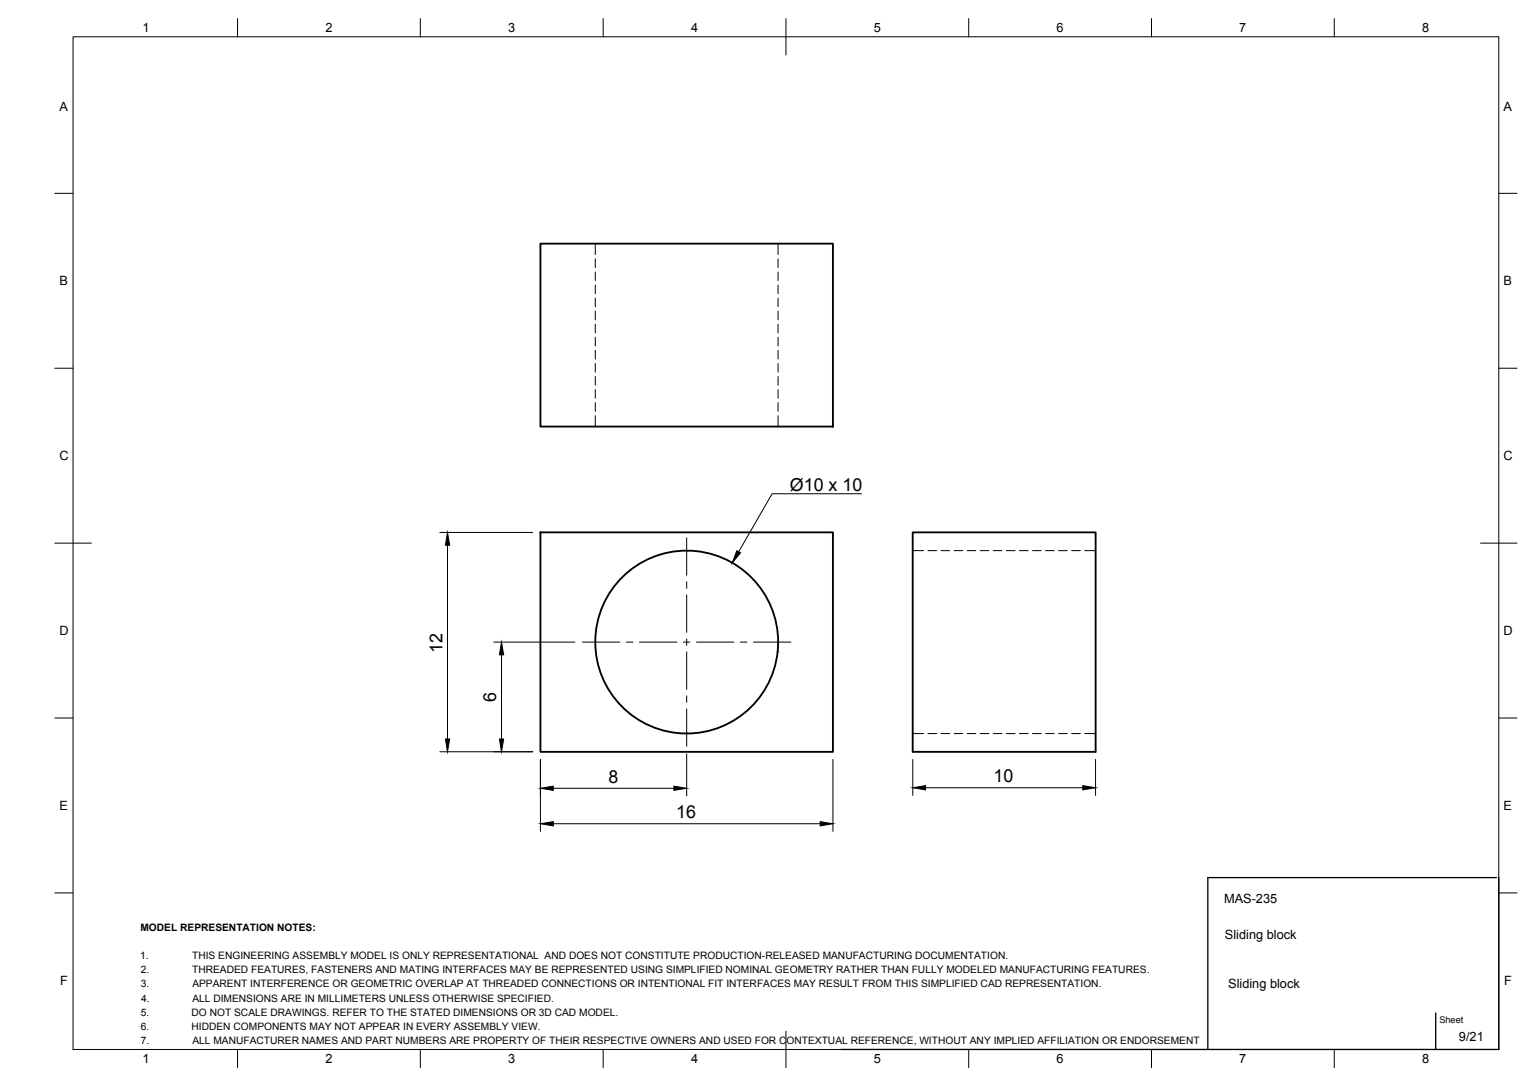
ISO-10303-21;
HEADER;
/* Generated by software containing ST-Developer
 * from STEP Tools, Inc. (www.steptools.com) 
 */

FILE_DESCRIPTION(
/* description */ ('Independent Whitworth quick-return mechanism. Crank radius40, ground-
center spacing80, lever180, connecting rod160, output guide X200. Nomi
nal stroke180 and long/short phase ratio2. Retained guide rods, replac
eable bearing sleeves and captured sliding shoe. No load or production
 rating assigned.'),
/* implementation_level */ '2;1');

FILE_NAME(
/* name */ 'Sliding block.step',
/* time_stamp */ '2026-11-09T18:22:56-08:00',
/* author */ (''),
/* organization */ (''),
/* preprocessor_version */ 'ST-DEVELOPER v20.2',
/* originating_system */ 'Autodesk Translation Framework v15.17.0.0',
/* authorisation */ '');

FILE_SCHEMA (('AUTOMOTIVE_DESIGN { 1 0 10303 214 3 1 1 }'));
ENDSEC;

DATA;
#10=MECHANICAL_DESIGN_GEOMETRIC_PRESENTATION_REPRESENTATION('',(#225),#4388);
#185=SHAPE_REPRESENTATION_RELATIONSHIP('SRR','None',#4484,#205);
#205=ADVANCED_BREP_SHAPE_REPRESENTATION('',(#245),#4374);
#225=STYLED_ITEM('',(#4592),#245);
#245=MANIFOLD_SOLID_BREP('Body1',#2330);
#281=FACE_BOUND('',#624,.T.);
#282=FACE_BOUND('',#626,.T.);
#343=PLANE('',#2660);
#344=PLANE('',#2661);
#345=PLANE('',#2662);
#346=PLANE('',#2663);
#347=PLANE('',#2664);
#348=PLANE('',#2665);
#449=FACE_OUTER_BOUND('',#618,.T.);
#450=FACE_OUTER_BOUND('',#619,.T.);
#451=FACE_OUTER_BOUND('',#620,.T.);
#452=FACE_OUTER_BOUND('',#621,.T.);
#453=FACE_OUTER_BOUND('',#622,.T.);
#454=FACE_OUTER_BOUND('',#623,.T.);
#455=FACE_OUTER_BOUND('',#625,.T.);
#618=EDGE_LOOP('',(#1786,#1787,#1788,#1789));
#619=EDGE_LOOP('',(#1790,#1791,#1792,#1793));
#620=EDGE_LOOP('',(#1794,#1795,#1796,#1797));
#621=EDGE_LOOP('',(#1798,#1799,#1800,#1801));
#622=EDGE_LOOP('',(#1802,#1803,#1804,#1805));
#623=EDGE_LOOP('',(#1806,#1807,#1808,#1809));
#624=EDGE_LOOP('',(#1810));
#625=EDGE_LOOP('',(#1811,#1812,#1813,#1814));
#626=EDGE_LOOP('',(#1815));
#815=LINE('',#3916,#954);
#816=LINE('',#3921,#955);
#817=LINE('',#3923,#956);
#818=LINE('',#3925,#957);
#819=LINE('',#3926,#958);
#820=LINE('',#3929,#959);
#821=LINE('',#3931,#960);
#822=LINE('',#3932,#961);
#823=LINE('',#3935,#962);
#824=LINE('',#3937,#963);
#825=LINE('',#3938,#964);
#826=LINE('',#3940,#965);
#827=LINE('',#3941,#966);
#954=VECTOR('',#3141,5.);
#955=VECTOR('',#3146,10.);
#956=VECTOR('',#3147,10.);
#957=VECTOR('',#3148,10.);
#958=VECTOR('',#3149,10.);
#959=VECTOR('',#3152,10.);
#960=VECTOR('',#3153,10.);
#961=VECTOR('',#3154,10.);
#962=VECTOR('',#3157,10.);
#963=VECTOR('',#3158,10.);
#964=VECTOR('',#3159,10.);
#965=VECTOR('',#3162,10.);
#966=VECTOR('',#3163,10.);
#1077=CIRCLE('',#2658,5.);
#1078=CIRCLE('',#2659,5.);
#1223=VERTEX_POINT('',#3913);
#1224=VERTEX_POINT('',#3915);
#1225=VERTEX_POINT('',#3919);
#1226=VERTEX_POINT('',#3920);
#1227=VERTEX_POINT('',#3922);
#1228=VERTEX_POINT('',#3924);
#1229=VERTEX_POINT('',#3928);
#1230=VERTEX_POINT('',#3930);
#1231=VERTEX_POINT('',#3934);
#1232=VERTEX_POINT('',#3936);
#1429=EDGE_CURVE('',#1223,#1223,#1077,.T.);
#1430=EDGE_CURVE('',#1223,#1224,#815,.T.);
#1431=EDGE_CURVE('',#1224,#1224,#1078,.T.);
#1432=EDGE_CURVE('',#1225,#1226,#816,.T.);
#1433=EDGE_CURVE('',#1226,#1227,#817,.T.);
#1434=EDGE_CURVE('',#1228,#1227,#818,.T.);
#1435=EDGE_CURVE('',#1225,#1228,#819,.T.);
#1436=EDGE_CURVE('',#1229,#1225,#820,.T.);
#1437=EDGE_CURVE('',#1230,#1228,#821,.T.);
#1438=EDGE_CURVE('',#1229,#1230,#822,.T.);
#1439=EDGE_CURVE('',#1231,#1229,#823,.T.);
#1440=EDGE_CURVE('',#1232,#1230,#824,.T.);
#1441=EDGE_CURVE('',#1231,#1232,#825,.T.);
#1442=EDGE_CURVE('',#1226,#1231,#826,.T.);
#1443=EDGE_CURVE('',#1227,#1232,#827,.T.);
#1786=ORIENTED_EDGE('',*,*,#1429,.F.);
#1787=ORIENTED_EDGE('',*,*,#1430,.T.);
#1788=ORIENTED_EDGE('',*,*,#1431,.F.);
#1789=ORIENTED_EDGE('',*,*,#1430,.F.);
#1790=ORIENTED_EDGE('',*,*,#1432,.T.);
#1791=ORIENTED_EDGE('',*,*,#1433,.T.);
#1792=ORIENTED_EDGE('',*,*,#1434,.F.);
#1793=ORIENTED_EDGE('',*,*,#1435,.F.);
#1794=ORIENTED_EDGE('',*,*,#1436,.T.);
#1795=ORIENTED_EDGE('',*,*,#1435,.T.);
#1796=ORIENTED_EDGE('',*,*,#1437,.F.);
#1797=ORIENTED_EDGE('',*,*,#1438,.F.);
#1798=ORIENTED_EDGE('',*,*,#1439,.T.);
#1799=ORIENTED_EDGE('',*,*,#1438,.T.);
#1800=ORIENTED_EDGE('',*,*,#1440,.F.);
#1801=ORIENTED_EDGE('',*,*,#1441,.F.);
#1802=ORIENTED_EDGE('',*,*,#1442,.T.);
#1803=ORIENTED_EDGE('',*,*,#1441,.T.);
#1804=ORIENTED_EDGE('',*,*,#1443,.F.);
#1805=ORIENTED_EDGE('',*,*,#1433,.F.);
#1806=ORIENTED_EDGE('',*,*,#1443,.T.);
#1807=ORIENTED_EDGE('',*,*,#1440,.T.);
#1808=ORIENTED_EDGE('',*,*,#1437,.T.);
#1809=ORIENTED_EDGE('',*,*,#1434,.T.);
#1810=ORIENTED_EDGE('',*,*,#1429,.T.);
#1811=ORIENTED_EDGE('',*,*,#1442,.F.);
#1812=ORIENTED_EDGE('',*,*,#1432,.F.);
#1813=ORIENTED_EDGE('',*,*,#1436,.F.);
#1814=ORIENTED_EDGE('',*,*,#1439,.F.);
#1815=ORIENTED_EDGE('',*,*,#1431,.T.);
#2136=CYLINDRICAL_SURFACE('',#2657,5.);
#2221=ADVANCED_FACE('',(#449),#2136,.F.);
#2222=ADVANCED_FACE('',(#450),#343,.T.);
#2223=ADVANCED_FACE('',(#451),#344,.T.);
#2224=ADVANCED_FACE('',(#452),#345,.T.);
#2225=ADVANCED_FACE('',(#453),#346,.T.);
#2226=ADVANCED_FACE('',(#454,#281),#347,.T.);
#2227=ADVANCED_FACE('',(#455,#282),#348,.F.);
#2330=CLOSED_SHELL('',(#2221,#2222,#2223,#2224,#2225,#2226,#2227));
#2656=AXIS2_PLACEMENT_3D('',#3911,#3135,#3136);
#2657=AXIS2_PLACEMENT_3D('',#3912,#3137,#3138);
#2658=AXIS2_PLACEMENT_3D('',#3914,#3139,#3140);
#2659=AXIS2_PLACEMENT_3D('',#3917,#3142,#3143);
#2660=AXIS2_PLACEMENT_3D('',#3918,#3144,#3145);
#2661=AXIS2_PLACEMENT_3D('',#3927,#3150,#3151);
#2662=AXIS2_PLACEMENT_3D('',#3933,#3155,#3156);
#2663=AXIS2_PLACEMENT_3D('',#3939,#3160,#3161);
#2664=AXIS2_PLACEMENT_3D('',#3942,#3164,#3165);
#2665=AXIS2_PLACEMENT_3D('',#3943,#3166,#3167);
#3135=DIRECTION('axis',(0.,0.,1.));
#3136=DIRECTION('refdir',(1.,0.,0.));
#3137=DIRECTION('center_axis',(0.,0.,-1.));
#3138=DIRECTION('ref_axis',(1.,0.,0.));
#3139=DIRECTION('center_axis',(0.,0.,-1.));
#3140=DIRECTION('ref_axis',(1.,0.,0.));
#3141=DIRECTION('',(0.,0.,-1.));
#3142=DIRECTION('center_axis',(0.,0.,1.));
#3143=DIRECTION('ref_axis',(1.,0.,0.));
#3144=DIRECTION('center_axis',(0.,1.,0.));
#3145=DIRECTION('ref_axis',(-1.,0.,0.));
#3146=DIRECTION('',(-1.,0.,0.));
#3147=DIRECTION('',(0.,0.,1.));
#3148=DIRECTION('',(-1.,0.,0.));
#3149=DIRECTION('',(0.,0.,1.));
#3150=DIRECTION('center_axis',(1.,0.,0.));
#3151=DIRECTION('ref_axis',(0.,1.,0.));
#3152=DIRECTION('',(0.,1.,0.));
#3153=DIRECTION('',(0.,1.,0.));
#3154=DIRECTION('',(0.,0.,1.));
#3155=DIRECTION('center_axis',(0.,-1.,0.));
#3156=DIRECTION('ref_axis',(1.,0.,0.));
#3157=DIRECTION('',(1.,0.,0.));
#3158=DIRECTION('',(1.,0.,0.));
#3159=DIRECTION('',(0.,0.,1.));
#3160=DIRECTION('center_axis',(-1.,0.,0.));
#3161=DIRECTION('ref_axis',(0.,-1.,0.));
#3162=DIRECTION('',(0.,-1.,0.));
#3163=DIRECTION('',(0.,-1.,0.));
#3164=DIRECTION('center_axis',(0.,0.,1.));
#3165=DIRECTION('ref_axis',(1.,0.,0.));
#3166=DIRECTION('center_axis',(0.,0.,1.));
#3167=DIRECTION('ref_axis',(1.,0.,0.));
#3911=CARTESIAN_POINT('',(0.,0.,0.));
#3912=CARTESIAN_POINT('Origin',(0.,0.,5.));
#3913=CARTESIAN_POINT('',(-5.,6.12323399573677E-16,10.));
#3914=CARTESIAN_POINT('Origin',(0.,0.,10.));
#3915=CARTESIAN_POINT('',(-5.,6.12323399573677E-16,0.));
#3916=CARTESIAN_POINT('',(-5.,6.12323399573677E-16,5.));
#3917=CARTESIAN_POINT('Origin',(0.,0.,0.));
#3918=CARTESIAN_POINT('Origin',(8.,6.,0.));
#3919=CARTESIAN_POINT('',(8.,6.,0.));
#3920=CARTESIAN_POINT('',(-8.,6.,0.));
#3921=CARTESIAN_POINT('',(8.,6.,0.));
#3922=CARTESIAN_POINT('',(-8.,6.,10.));
#3923=CARTESIAN_POINT('',(-8.,6.,0.));
#3924=CARTESIAN_POINT('',(8.,6.,10.));
#3925=CARTESIAN_POINT('',(8.,6.,10.));
#3926=CARTESIAN_POINT('',(8.,6.,0.));
#3927=CARTESIAN_POINT('Origin',(8.,-6.,0.));
#3928=CARTESIAN_POINT('',(8.,-6.,0.));
#3929=CARTESIAN_POINT('',(8.,-6.,0.));
#3930=CARTESIAN_POINT('',(8.,-6.,10.));
#3931=CARTESIAN_POINT('',(8.,-6.,10.));
#3932=CARTESIAN_POINT('',(8.,-6.,0.));
#3933=CARTESIAN_POINT('Origin',(-8.,-6.,0.));
#3934=CARTESIAN_POINT('',(-8.,-6.,0.));
#3935=CARTESIAN_POINT('',(-8.,-6.,0.));
#3936=CARTESIAN_POINT('',(-8.,-6.,10.));
#3937=CARTESIAN_POINT('',(-8.,-6.,10.));
#3938=CARTESIAN_POINT('',(-8.,-6.,0.));
#3939=CARTESIAN_POINT('Origin',(-8.,6.,0.));
#3940=CARTESIAN_POINT('',(-8.,6.,0.));
#3941=CARTESIAN_POINT('',(-8.,6.,10.));
#3942=CARTESIAN_POINT('Origin',(0.,0.,10.));
#3943=CARTESIAN_POINT('Origin',(0.,0.,0.));
#4352=UNCERTAINTY_MEASURE_WITH_UNIT(LENGTH_MEASURE(0.01),#4389,
'DISTANCE_ACCURACY_VALUE',
'Maximum model space distance between geometric entities at asserted c
onnectivities');
#4366=UNCERTAINTY_MEASURE_WITH_UNIT(LENGTH_MEASURE(0.01),#4389,
'DISTANCE_ACCURACY_VALUE',
'Maximum model space distance between geometric entities at asserted c
onnectivities');
#4374=(
GEOMETRIC_REPRESENTATION_CONTEXT(3)
GLOBAL_UNCERTAINTY_ASSIGNED_CONTEXT((#4352))
GLOBAL_UNIT_ASSIGNED_CONTEXT((#4389,#4391,#4392))
REPRESENTATION_CONTEXT('','3D')
);
#4388=(
GEOMETRIC_REPRESENTATION_CONTEXT(3)
GLOBAL_UNCERTAINTY_ASSIGNED_CONTEXT((#4366))
GLOBAL_UNIT_ASSIGNED_CONTEXT((#4389,#4391,#4392))
REPRESENTATION_CONTEXT('','3D')
);
#4389=(
LENGTH_UNIT()
NAMED_UNIT(*)
SI_UNIT(.MILLI.,.METRE.)
);
#4391=(
NAMED_UNIT(*)
PLANE_ANGLE_UNIT()
SI_UNIT($,.RADIAN.)
);
#4392=(
NAMED_UNIT(*)
SI_UNIT($,.STERADIAN.)
SOLID_ANGLE_UNIT()
);
#4400=SHAPE_DEFINITION_REPRESENTATION(#4421,#4484);
#4421=PRODUCT_DEFINITION_SHAPE('',$,#4506);
#4484=SHAPE_REPRESENTATION('',(#2656),#4374);
#4498=PRODUCT_DEFINITION_CONTEXT('part definition',#4563,'design');
#4506=PRODUCT_DEFINITION('Sliding block','Sliding block',#4527,#4498);
#4527=PRODUCT_DEFINITION_FORMATION('',$,#4572);
#4563=APPLICATION_CONTEXT(
'Core Data for Automotive Mechanical Design Process');
#4564=PRODUCT_CONTEXT('part definition',#4563,'mechanical');
#4572=PRODUCT('Sliding block','Sliding block',$,(#4564));
#4592=PRESENTATION_STYLE_ASSIGNMENT((#4606));
#4606=SURFACE_STYLE_USAGE(.BOTH.,#4620);
#4620=SURFACE_SIDE_STYLE('',(#4634));
#4634=SURFACE_STYLE_FILL_AREA(#4648);
#4648=FILL_AREA_STYLE('Shoe gray',(#4662));
#4662=FILL_AREA_STYLE_COLOUR('Shoe gray',#4676);
#4676=COLOUR_RGB('Shoe gray',0.407843137254902,0.447058823529412,0.498039215686275);
ENDSEC;
END-ISO-10303-21;
